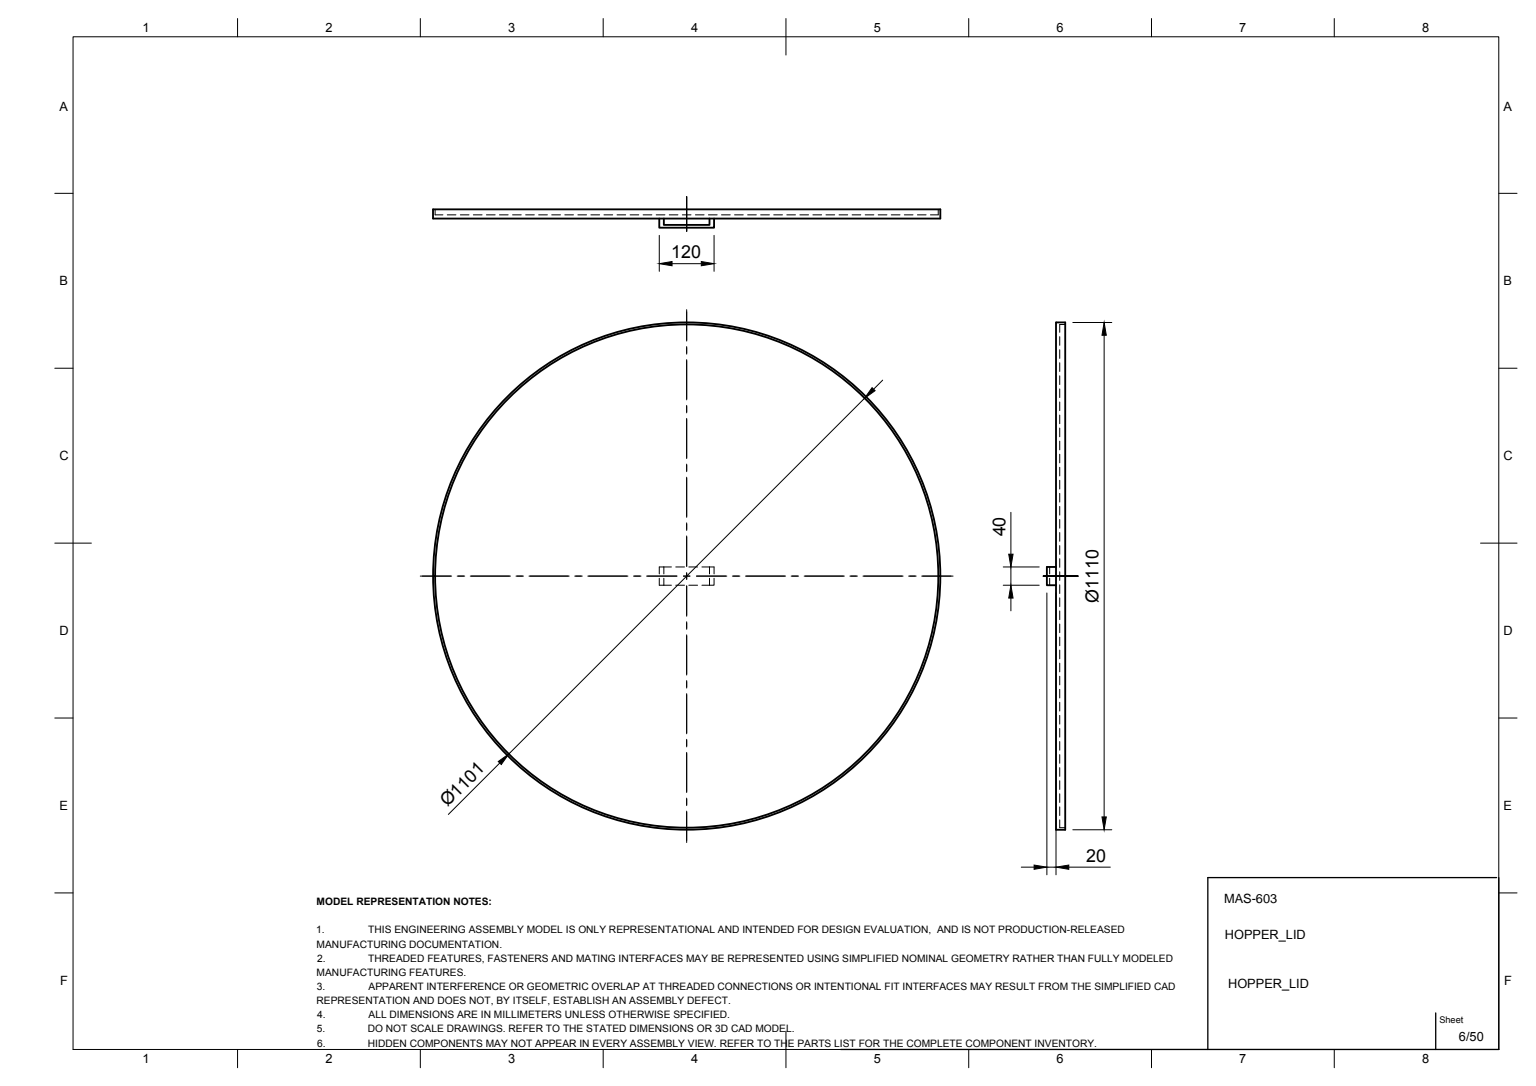
ISO-10303-21;
HEADER;
FILE_DESCRIPTION((''),'2;1');
FILE_NAME('HOPPER_LID.step','2026-10-01T22:06:14-07:00',(''),(''),'','','');
FILE_SCHEMA (('AUTOMOTIVE_DESIGN { 1 0 10303 214 3 1 1 }'));
ENDSEC;
DATA;
#10=MECHANICAL_DESIGN_GEOMETRIC_PRESENTATION_REPRESENTATION('',(#982),#50440);
#892=SHAPE_REPRESENTATION_RELATIONSHIP('SRR','None',#50622,#937) ;
#937=ADVANCED_BREP_SHAPE_REPRESENTATION('',(#1038),#50391) ;
#982=STYLED_ITEM('',(#50884),#1038) ;
#1038=MANIFOLD_SOLID_BREP('HOPPER_LID',#28630) ;
#1127=FACE_BOUND('',#3985,.T.) ;
#1128=FACE_BOUND('',#3989,.T.) ;
#1129=FACE_BOUND('',#3990,.T.) ;
#1467=PLANE('',#29313) ;
#1468=PLANE('',#29314) ;
#1469=PLANE('',#29315) ;
#1470=PLANE('',#29316) ;
#1471=PLANE('',#29317) ;
#1472=PLANE('',#29318) ;
#1473=PLANE('',#29319) ;
#1474=PLANE('',#29320) ;
#1475=PLANE('',#29324) ;
#1476=PLANE('',#29328) ;
#1477=PLANE('',#29329) ;
#2406=FACE_OUTER_BOUND('',#3975,.T.) ;
#2407=FACE_OUTER_BOUND('',#3976,.T.) ;
#2408=FACE_OUTER_BOUND('',#3977,.T.) ;
#2409=FACE_OUTER_BOUND('',#3978,.T.) ;
#2410=FACE_OUTER_BOUND('',#3979,.T.) ;
#2411=FACE_OUTER_BOUND('',#3980,.T.) ;
#2412=FACE_OUTER_BOUND('',#3981,.T.) ;
#2413=FACE_OUTER_BOUND('',#3982,.T.) ;
#2414=FACE_OUTER_BOUND('',#3983,.T.) ;
#2415=FACE_OUTER_BOUND('',#3984,.T.) ;
#2416=FACE_OUTER_BOUND('',#3986,.T.) ;
#2417=FACE_OUTER_BOUND('',#3987,.T.) ;
#2418=FACE_OUTER_BOUND('',#3988,.T.) ;
#3975=EDGE_LOOP('',(#18917,#18918,#18919,#18920)) ;
#3976=EDGE_LOOP('',(#18921,#18922,#18923,#18924)) ;
#3977=EDGE_LOOP('',(#18925,#18926,#18927,#18928)) ;
#3978=EDGE_LOOP('',(#18929,#18930,#18931,#18932,#18933,#18934,#18935,#18936)) ;
#3979=EDGE_LOOP('',(#18937,#18938,#18939,#18940,#18941,#18942,#18943,#18944)) ;
#3980=EDGE_LOOP('',(#18945,#18946,#18947,#18948)) ;
#3981=EDGE_LOOP('',(#18949,#18950,#18951,#18952)) ;
#3982=EDGE_LOOP('',(#18953,#18954,#18955,#18956)) ;
#3983=EDGE_LOOP('',(#18957,#18958,#18959,#18960)) ;
#3984=EDGE_LOOP('',(#18961)) ;
#3985=EDGE_LOOP('',(#18962)) ;
#3986=EDGE_LOOP('',(#18963,#18964,#18965,#18966)) ;
#3987=EDGE_LOOP('',(#18967)) ;
#3988=EDGE_LOOP('',(#18968)) ;
#3989=EDGE_LOOP('',(#18969,#18970,#18971,#18972)) ;
#3990=EDGE_LOOP('',(#18973,#18974,#18975,#18976)) ;
#5859=LINE('',#41599,#8331) ;
#5860=LINE('',#41601,#8332) ;
#5861=LINE('',#41603,#8333) ;
#5862=LINE('',#41604,#8334) ;
#5863=LINE('',#41607,#8335) ;
#5864=LINE('',#41609,#8336) ;
#5865=LINE('',#41610,#8337) ;
#5866=LINE('',#41613,#8338) ;
#5867=LINE('',#41615,#8339) ;
#5868=LINE('',#41616,#8340) ;
#5869=LINE('',#41619,#8341) ;
#5870=LINE('',#41621,#8342) ;
#5871=LINE('',#41623,#8343) ;
#5872=LINE('',#41625,#8344) ;
#5873=LINE('',#41626,#8345) ;
#5874=LINE('',#41629,#8346) ;
#5875=LINE('',#41631,#8347) ;
#5876=LINE('',#41633,#8348) ;
#5877=LINE('',#41635,#8349) ;
#5878=LINE('',#41636,#8350) ;
#5879=LINE('',#41638,#8351) ;
#5880=LINE('',#41639,#8352) ;
#5881=LINE('',#41641,#8353) ;
#5882=LINE('',#41643,#8354) ;
#5883=LINE('',#41648,#8355) ;
#5884=LINE('',#41656,#8356) ;
#8331=VECTOR('',#32712,1.) ;
#8332=VECTOR('',#32713,1.) ;
#8333=VECTOR('',#32714,1.) ;
#8334=VECTOR('',#32715,1.) ;
#8335=VECTOR('',#32718,1.) ;
#8336=VECTOR('',#32719,1.) ;
#8337=VECTOR('',#32720,1.) ;
#8338=VECTOR('',#32723,1.) ;
#8339=VECTOR('',#32724,1.) ;
#8340=VECTOR('',#32725,1.) ;
#8341=VECTOR('',#32728,1.) ;
#8342=VECTOR('',#32729,1.) ;
#8343=VECTOR('',#32730,1.) ;
#8344=VECTOR('',#32731,1.) ;
#8345=VECTOR('',#32732,1.) ;
#8346=VECTOR('',#32735,1.) ;
#8347=VECTOR('',#32736,1.) ;
#8348=VECTOR('',#32737,1.) ;
#8349=VECTOR('',#32738,1.) ;
#8350=VECTOR('',#32739,1.) ;
#8351=VECTOR('',#32742,1.) ;
#8352=VECTOR('',#32743,1.) ;
#8353=VECTOR('',#32746,1.) ;
#8354=VECTOR('',#32749,1.) ;
#8355=VECTOR('',#32754,55.05) ;
#8356=VECTOR('',#32765,55.5) ;
#10720=CIRCLE('',#29322,55.05) ;
#10721=CIRCLE('',#29323,55.05) ;
#10722=CIRCLE('',#29325,55.5) ;
#10723=CIRCLE('',#29327,55.5) ;
#11963=VERTEX_POINT('',#41597) ;
#11964=VERTEX_POINT('',#41598) ;
#11965=VERTEX_POINT('',#41600) ;
#11966=VERTEX_POINT('',#41602) ;
#11967=VERTEX_POINT('',#41606) ;
#11968=VERTEX_POINT('',#41608) ;
#11969=VERTEX_POINT('',#41612) ;
#11970=VERTEX_POINT('',#41614) ;
#11971=VERTEX_POINT('',#41618) ;
#11972=VERTEX_POINT('',#41620) ;
#11973=VERTEX_POINT('',#41622) ;
#11974=VERTEX_POINT('',#41624) ;
#11975=VERTEX_POINT('',#41628) ;
#11976=VERTEX_POINT('',#41630) ;
#11977=VERTEX_POINT('',#41632) ;
#11978=VERTEX_POINT('',#41634) ;
#11979=VERTEX_POINT('',#41645) ;
#11980=VERTEX_POINT('',#41647) ;
#11981=VERTEX_POINT('',#41651) ;
#11982=VERTEX_POINT('',#41654) ;
#14724=EDGE_CURVE('',#11963,#11964,#5859,.T.) ;
#14725=EDGE_CURVE('',#11965,#11963,#5860,.T.) ;
#14726=EDGE_CURVE('',#11966,#11965,#5861,.T.) ;
#14727=EDGE_CURVE('',#11964,#11966,#5862,.T.) ;
#14728=EDGE_CURVE('',#11964,#11967,#5863,.T.) ;
#14729=EDGE_CURVE('',#11968,#11966,#5864,.T.) ;
#14730=EDGE_CURVE('',#11968,#11967,#5865,.T.) ;
#14731=EDGE_CURVE('',#11969,#11963,#5866,.T.) ;
#14732=EDGE_CURVE('',#11969,#11970,#5867,.T.) ;
#14733=EDGE_CURVE('',#11965,#11970,#5868,.T.) ;
#14734=EDGE_CURVE('',#11971,#11967,#5869,.T.) ;
#14735=EDGE_CURVE('',#11972,#11971,#5870,.T.) ;
#14736=EDGE_CURVE('',#11973,#11972,#5871,.T.) ;
#14737=EDGE_CURVE('',#11973,#11974,#5872,.T.) ;
#14738=EDGE_CURVE('',#11969,#11974,#5873,.T.) ;
#14739=EDGE_CURVE('',#11975,#11970,#5874,.T.) ;
#14740=EDGE_CURVE('',#11976,#11975,#5875,.T.) ;
#14741=EDGE_CURVE('',#11977,#11976,#5876,.T.) ;
#14742=EDGE_CURVE('',#11977,#11978,#5877,.T.) ;
#14743=EDGE_CURVE('',#11968,#11978,#5878,.T.) ;
#14744=EDGE_CURVE('',#11976,#11973,#5879,.T.) ;
#14745=EDGE_CURVE('',#11972,#11977,#5880,.T.) ;
#14746=EDGE_CURVE('',#11978,#11971,#5881,.T.) ;
#14747=EDGE_CURVE('',#11974,#11975,#5882,.T.) ;
#14748=EDGE_CURVE('',#11979,#11979,#10720,.T.) ;
#14749=EDGE_CURVE('',#11979,#11980,#5883,.T.) ;
#14750=EDGE_CURVE('',#11980,#11980,#10721,.T.) ;
#14751=EDGE_CURVE('',#11981,#11981,#10722,.T.) ;
#14752=EDGE_CURVE('',#11982,#11982,#10723,.T.) ;
#14753=EDGE_CURVE('',#11982,#11981,#5884,.T.) ;
#18917=ORIENTED_EDGE('',*,*,#14724,.F.) ;
#18918=ORIENTED_EDGE('',*,*,#14725,.F.) ;
#18919=ORIENTED_EDGE('',*,*,#14726,.F.) ;
#18920=ORIENTED_EDGE('',*,*,#14727,.F.) ;
#18921=ORIENTED_EDGE('',*,*,#14728,.F.) ;
#18922=ORIENTED_EDGE('',*,*,#14727,.T.) ;
#18923=ORIENTED_EDGE('',*,*,#14729,.F.) ;
#18924=ORIENTED_EDGE('',*,*,#14730,.T.) ;
#18925=ORIENTED_EDGE('',*,*,#14731,.F.) ;
#18926=ORIENTED_EDGE('',*,*,#14732,.T.) ;
#18927=ORIENTED_EDGE('',*,*,#14733,.F.) ;
#18928=ORIENTED_EDGE('',*,*,#14725,.T.) ;
#18929=ORIENTED_EDGE('',*,*,#14731,.T.) ;
#18930=ORIENTED_EDGE('',*,*,#14724,.T.) ;
#18931=ORIENTED_EDGE('',*,*,#14728,.T.) ;
#18932=ORIENTED_EDGE('',*,*,#14734,.F.) ;
#18933=ORIENTED_EDGE('',*,*,#14735,.F.) ;
#18934=ORIENTED_EDGE('',*,*,#14736,.F.) ;
#18935=ORIENTED_EDGE('',*,*,#14737,.T.) ;
#18936=ORIENTED_EDGE('',*,*,#14738,.F.) ;
#18937=ORIENTED_EDGE('',*,*,#14729,.T.) ;
#18938=ORIENTED_EDGE('',*,*,#14726,.T.) ;
#18939=ORIENTED_EDGE('',*,*,#14733,.T.) ;
#18940=ORIENTED_EDGE('',*,*,#14739,.F.) ;
#18941=ORIENTED_EDGE('',*,*,#14740,.F.) ;
#18942=ORIENTED_EDGE('',*,*,#14741,.F.) ;
#18943=ORIENTED_EDGE('',*,*,#14742,.T.) ;
#18944=ORIENTED_EDGE('',*,*,#14743,.F.) ;
#18945=ORIENTED_EDGE('',*,*,#14744,.T.) ;
#18946=ORIENTED_EDGE('',*,*,#14736,.T.) ;
#18947=ORIENTED_EDGE('',*,*,#14745,.T.) ;
#18948=ORIENTED_EDGE('',*,*,#14741,.T.) ;
#18949=ORIENTED_EDGE('',*,*,#14735,.T.) ;
#18950=ORIENTED_EDGE('',*,*,#14746,.F.) ;
#18951=ORIENTED_EDGE('',*,*,#14742,.F.) ;
#18952=ORIENTED_EDGE('',*,*,#14745,.F.) ;
#18953=ORIENTED_EDGE('',*,*,#14740,.T.) ;
#18954=ORIENTED_EDGE('',*,*,#14747,.F.) ;
#18955=ORIENTED_EDGE('',*,*,#14737,.F.) ;
#18956=ORIENTED_EDGE('',*,*,#14744,.F.) ;
#18957=ORIENTED_EDGE('',*,*,#14748,.F.) ;
#18958=ORIENTED_EDGE('',*,*,#14749,.T.) ;
#18959=ORIENTED_EDGE('',*,*,#14750,.F.) ;
#18960=ORIENTED_EDGE('',*,*,#14749,.F.) ;
#18961=ORIENTED_EDGE('',*,*,#14751,.T.) ;
#18962=ORIENTED_EDGE('',*,*,#14748,.T.) ;
#18963=ORIENTED_EDGE('',*,*,#14752,.F.) ;
#18964=ORIENTED_EDGE('',*,*,#14753,.T.) ;
#18965=ORIENTED_EDGE('',*,*,#14751,.F.) ;
#18966=ORIENTED_EDGE('',*,*,#14753,.F.) ;
#18967=ORIENTED_EDGE('',*,*,#14750,.T.) ;
#18968=ORIENTED_EDGE('',*,*,#14752,.T.) ;
#18969=ORIENTED_EDGE('',*,*,#14738,.T.) ;
#18970=ORIENTED_EDGE('',*,*,#14747,.T.) ;
#18971=ORIENTED_EDGE('',*,*,#14739,.T.) ;
#18972=ORIENTED_EDGE('',*,*,#14732,.F.) ;
#18973=ORIENTED_EDGE('',*,*,#14730,.F.) ;
#18974=ORIENTED_EDGE('',*,*,#14743,.T.) ;
#18975=ORIENTED_EDGE('',*,*,#14746,.T.) ;
#18976=ORIENTED_EDGE('',*,*,#14734,.T.) ;
#26656=CYLINDRICAL_SURFACE('',#29321,55.05) ;
#26657=CYLINDRICAL_SURFACE('',#29326,55.5) ;
#27141=ADVANCED_FACE('',(#2406),#1467,.F.) ;
#27142=ADVANCED_FACE('',(#2407),#1468,.T.) ;
#27143=ADVANCED_FACE('',(#2408),#1469,.T.) ;
#27144=ADVANCED_FACE('',(#2409),#1470,.F.) ;
#27145=ADVANCED_FACE('',(#2410),#1471,.F.) ;
#27146=ADVANCED_FACE('',(#2411),#1472,.T.) ;
#27147=ADVANCED_FACE('',(#2412),#1473,.F.) ;
#27148=ADVANCED_FACE('',(#2413),#1474,.F.) ;
#27149=ADVANCED_FACE('',(#2414),#26656,.F.) ;
#27150=ADVANCED_FACE('',(#2415,#1127),#1475,.T.) ;
#27151=ADVANCED_FACE('',(#2416),#26657,.T.) ;
#27152=ADVANCED_FACE('',(#2417),#1476,.T.) ;
#27153=ADVANCED_FACE('',(#2418,#1128,#1129),#1477,.T.) ;
#28630=CLOSED_SHELL('',(#27141,#27142,#27143,#27144,#27145,#27146,#27147,
#27148,#27149,#27150,#27151,#27152,#27153)) ;
#29312=AXIS2_PLACEMENT_3D('',#41595,#32708,#32709) ;
#29313=AXIS2_PLACEMENT_3D('',#41596,#32710,#32711) ;
#29314=AXIS2_PLACEMENT_3D('',#41605,#32716,#32717) ;
#29315=AXIS2_PLACEMENT_3D('',#41611,#32721,#32722) ;
#29316=AXIS2_PLACEMENT_3D('',#41617,#32726,#32727) ;
#29317=AXIS2_PLACEMENT_3D('',#41627,#32733,#32734) ;
#29318=AXIS2_PLACEMENT_3D('',#41637,#32740,#32741) ;
#29319=AXIS2_PLACEMENT_3D('',#41640,#32744,#32745) ;
#29320=AXIS2_PLACEMENT_3D('',#41642,#32747,#32748) ;
#29321=AXIS2_PLACEMENT_3D('',#41644,#32750,#32751) ;
#29322=AXIS2_PLACEMENT_3D('',#41646,#32752,#32753) ;
#29323=AXIS2_PLACEMENT_3D('',#41649,#32755,#32756) ;
#29324=AXIS2_PLACEMENT_3D('',#41650,#32757,#32758) ;
#29325=AXIS2_PLACEMENT_3D('',#41652,#32759,#32760) ;
#29326=AXIS2_PLACEMENT_3D('',#41653,#32761,#32762) ;
#29327=AXIS2_PLACEMENT_3D('',#41655,#32763,#32764) ;
#29328=AXIS2_PLACEMENT_3D('',#41657,#32766,#32767) ;
#29329=AXIS2_PLACEMENT_3D('',#41658,#32768,#32769) ;
#32708=DIRECTION('axis',(0.,0.,1.)) ;
#32709=DIRECTION('refdir',(1.,0.,0.)) ;
#32710=DIRECTION('center_axis',(0.,0.,1.)) ;
#32711=DIRECTION('ref_axis',(1.,0.,0.)) ;
#32712=DIRECTION('',(-1.,0.,0.)) ;
#32713=DIRECTION('',(0.,1.,0.)) ;
#32714=DIRECTION('',(1.,0.,0.)) ;
#32715=DIRECTION('',(0.,-1.,0.)) ;
#32716=DIRECTION('center_axis',(1.,0.,0.)) ;
#32717=DIRECTION('ref_axis',(0.,0.,-1.)) ;
#32718=DIRECTION('',(0.,0.,-1.)) ;
#32719=DIRECTION('',(0.,0.,1.)) ;
#32720=DIRECTION('',(0.,1.,0.)) ;
#32721=DIRECTION('center_axis',(-1.,0.,0.)) ;
#32722=DIRECTION('ref_axis',(0.,0.,1.)) ;
#32723=DIRECTION('',(0.,0.,1.)) ;
#32724=DIRECTION('',(0.,-1.,0.)) ;
#32725=DIRECTION('',(0.,0.,-1.)) ;
#32726=DIRECTION('center_axis',(0.,-1.,0.)) ;
#32727=DIRECTION('ref_axis',(0.,0.,-1.)) ;
#32728=DIRECTION('',(1.,0.,0.)) ;
#32729=DIRECTION('',(0.,0.,-1.)) ;
#32730=DIRECTION('',(-1.,0.,0.)) ;
#32731=DIRECTION('',(0.,0.,-1.)) ;
#32732=DIRECTION('',(1.,0.,0.)) ;
#32733=DIRECTION('center_axis',(0.,1.,0.)) ;
#32734=DIRECTION('ref_axis',(0.,0.,1.)) ;
#32735=DIRECTION('',(-1.,0.,0.)) ;
#32736=DIRECTION('',(0.,0.,-1.)) ;
#32737=DIRECTION('',(1.,0.,0.)) ;
#32738=DIRECTION('',(0.,0.,-1.)) ;
#32739=DIRECTION('',(-1.,0.,0.)) ;
#32740=DIRECTION('center_axis',(0.,0.,1.)) ;
#32741=DIRECTION('ref_axis',(1.,0.,0.)) ;
#32742=DIRECTION('',(0.,1.,0.)) ;
#32743=DIRECTION('',(0.,-1.,0.)) ;
#32744=DIRECTION('center_axis',(1.,0.,0.)) ;
#32745=DIRECTION('ref_axis',(0.,0.,-1.)) ;
#32746=DIRECTION('',(0.,1.,0.)) ;
#32747=DIRECTION('center_axis',(-1.,0.,0.)) ;
#32748=DIRECTION('ref_axis',(0.,0.,1.)) ;
#32749=DIRECTION('',(0.,-1.,0.)) ;
#32750=DIRECTION('center_axis',(0.,0.,1.)) ;
#32751=DIRECTION('ref_axis',(1.,0.,0.)) ;
#32752=DIRECTION('center_axis',(0.,0.,1.)) ;
#32753=DIRECTION('ref_axis',(1.,0.,0.)) ;
#32754=DIRECTION('',(0.,0.,1.)) ;
#32755=DIRECTION('center_axis',(0.,0.,-1.)) ;
#32756=DIRECTION('ref_axis',(1.,0.,0.)) ;
#32757=DIRECTION('center_axis',(0.,0.,-1.)) ;
#32758=DIRECTION('ref_axis',(-1.,0.,0.)) ;
#32759=DIRECTION('center_axis',(0.,0.,-1.)) ;
#32760=DIRECTION('ref_axis',(1.,0.,0.)) ;
#32761=DIRECTION('center_axis',(0.,0.,1.)) ;
#32762=DIRECTION('ref_axis',(1.,0.,0.)) ;
#32763=DIRECTION('center_axis',(0.,0.,1.)) ;
#32764=DIRECTION('ref_axis',(1.,0.,0.)) ;
#32765=DIRECTION('',(0.,0.,-1.)) ;
#32766=DIRECTION('center_axis',(0.,0.,-1.)) ;
#32767=DIRECTION('ref_axis',(-1.,0.,0.)) ;
#32768=DIRECTION('center_axis',(0.,0.,1.)) ;
#32769=DIRECTION('ref_axis',(1.,0.,0.)) ;
#41595=CARTESIAN_POINT('',(0.,0.,0.)) ;
#41596=CARTESIAN_POINT('Origin',(0.,0.,113.4)) ;
#41597=CARTESIAN_POINT('',(5.,2.,113.4)) ;
#41598=CARTESIAN_POINT('',(-5.,2.,113.4)) ;
#41599=CARTESIAN_POINT('',(0.,2.,113.4)) ;
#41600=CARTESIAN_POINT('',(5.,-2.,113.4)) ;
#41601=CARTESIAN_POINT('',(5.,0.,113.4)) ;
#41602=CARTESIAN_POINT('',(-5.,-2.,113.4)) ;
#41603=CARTESIAN_POINT('',(0.,-2.,113.4)) ;
#41604=CARTESIAN_POINT('',(-5.,0.,113.4)) ;
#41605=CARTESIAN_POINT('Origin',(-5.,0.,112.7)) ;
#41606=CARTESIAN_POINT('',(-5.,2.,112.)) ;
#41607=CARTESIAN_POINT('',(-5.,2.,112.85)) ;
#41608=CARTESIAN_POINT('',(-5.,-2.,112.)) ;
#41609=CARTESIAN_POINT('',(-5.,-2.,112.85)) ;
#41610=CARTESIAN_POINT('',(-5.,0.,112.)) ;
#41611=CARTESIAN_POINT('Origin',(5.,0.,112.7)) ;
#41612=CARTESIAN_POINT('',(5.,2.,112.)) ;
#41613=CARTESIAN_POINT('',(5.,2.,112.85)) ;
#41614=CARTESIAN_POINT('',(5.,-2.,112.)) ;
#41615=CARTESIAN_POINT('',(5.,0.,112.)) ;
#41616=CARTESIAN_POINT('',(5.,-2.,112.85)) ;
#41617=CARTESIAN_POINT('Origin',(0.,2.,113.)) ;
#41618=CARTESIAN_POINT('',(-6.,2.,112.)) ;
#41619=CARTESIAN_POINT('',(0.,2.,112.)) ;
#41620=CARTESIAN_POINT('',(-6.,2.,114.)) ;
#41621=CARTESIAN_POINT('',(-6.,2.,113.)) ;
#41622=CARTESIAN_POINT('',(6.,2.,114.)) ;
#41623=CARTESIAN_POINT('',(0.,2.,114.)) ;
#41624=CARTESIAN_POINT('',(6.,2.,112.)) ;
#41625=CARTESIAN_POINT('',(6.,2.,113.)) ;
#41626=CARTESIAN_POINT('',(0.,2.,112.)) ;
#41627=CARTESIAN_POINT('Origin',(0.,-2.,113.)) ;
#41628=CARTESIAN_POINT('',(6.,-2.,112.)) ;
#41629=CARTESIAN_POINT('',(0.,-2.,112.)) ;
#41630=CARTESIAN_POINT('',(6.,-2.,114.)) ;
#41631=CARTESIAN_POINT('',(6.,-2.,113.)) ;
#41632=CARTESIAN_POINT('',(-6.,-2.,114.)) ;
#41633=CARTESIAN_POINT('',(0.,-2.,114.)) ;
#41634=CARTESIAN_POINT('',(-6.,-2.,112.)) ;
#41635=CARTESIAN_POINT('',(-6.,-2.,113.)) ;
#41636=CARTESIAN_POINT('',(0.,-2.,112.)) ;
#41637=CARTESIAN_POINT('Origin',(0.,0.,114.)) ;
#41638=CARTESIAN_POINT('',(6.,0.,114.)) ;
#41639=CARTESIAN_POINT('',(-6.,0.,114.)) ;
#41640=CARTESIAN_POINT('Origin',(-6.,0.,113.)) ;
#41641=CARTESIAN_POINT('',(-6.,0.,112.)) ;
#41642=CARTESIAN_POINT('Origin',(6.,0.,113.)) ;
#41643=CARTESIAN_POINT('',(6.,0.,112.)) ;
#41644=CARTESIAN_POINT('Origin',(0.,0.,110.6)) ;
#41645=CARTESIAN_POINT('',(-55.05,-6.74168062930618E-15,110.)) ;
#41646=CARTESIAN_POINT('Origin',(0.,0.,110.)) ;
#41647=CARTESIAN_POINT('',(-55.05,6.74168062930618E-15,111.2)) ;
#41648=CARTESIAN_POINT('',(-55.05,-6.74168062930618E-15,110.6)) ;
#41649=CARTESIAN_POINT('Origin',(0.,0.,111.2)) ;
#41650=CARTESIAN_POINT('Origin',(0.,0.,110.)) ;
#41651=CARTESIAN_POINT('',(-55.5,-6.79678973526781E-15,110.)) ;
#41652=CARTESIAN_POINT('Origin',(0.,0.,110.)) ;
#41653=CARTESIAN_POINT('Origin',(0.,0.,111.6)) ;
#41654=CARTESIAN_POINT('',(-55.5,-6.79678973526781E-15,112.)) ;
#41655=CARTESIAN_POINT('Origin',(0.,0.,112.)) ;
#41656=CARTESIAN_POINT('',(-55.5,-6.79678973526781E-15,111.6)) ;
#41657=CARTESIAN_POINT('Origin',(0.,0.,111.2)) ;
#41658=CARTESIAN_POINT('Origin',(0.,0.,112.)) ;
#50338=UNCERTAINTY_MEASURE_WITH_UNIT(LENGTH_MEASURE(0.001),#50441,
'DISTANCE_ACCURACY_VALUE',
'Maximum model space distance between geometric entities at asserted c
onnectivities') ;
#50387=UNCERTAINTY_MEASURE_WITH_UNIT(LENGTH_MEASURE(0.001),#50441,
'DISTANCE_ACCURACY_VALUE',
'Maximum model space distance between geometric entities at asserted c
onnectivities') ;
#50391=(
GEOMETRIC_REPRESENTATION_CONTEXT(3)
GLOBAL_UNCERTAINTY_ASSIGNED_CONTEXT((#50338))
GLOBAL_UNIT_ASSIGNED_CONTEXT((#50441,#50443,#50444))
REPRESENTATION_CONTEXT('','3D')
) ;
#50440=(
GEOMETRIC_REPRESENTATION_CONTEXT(3)
GLOBAL_UNCERTAINTY_ASSIGNED_CONTEXT((#50387))
GLOBAL_UNIT_ASSIGNED_CONTEXT((#50441,#50443,#50444))
REPRESENTATION_CONTEXT('','3D')
) ;
#50441=(
LENGTH_UNIT()
NAMED_UNIT(*)
SI_UNIT(.CENTI.,.METRE.)
) ;
#50443=(
NAMED_UNIT(*)
PLANE_ANGLE_UNIT()
SI_UNIT($,.RADIAN.)
) ;
#50444=(
NAMED_UNIT(*)
SI_UNIT($,.STERADIAN.)
SOLID_ANGLE_UNIT()
) ;
#50448=SHAPE_DEFINITION_REPRESENTATION(#50500,#50622) ;
#50500=PRODUCT_DEFINITION_SHAPE('',$,#50675) ;
#50622=SHAPE_REPRESENTATION('',(#29312),#50391) ;
#50671=PRODUCT_DEFINITION_CONTEXT('part definition',#50829,'design') ;
#50675=PRODUCT_DEFINITION('HOPPER_LID','HOPPER_LID',#50727,
#50671) ;
#50727=PRODUCT_DEFINITION_FORMATION('',$,#50834) ;
#50829=APPLICATION_CONTEXT(
'Core Data for Automotive Mechanical Design Process') ;
#50830=PRODUCT_CONTEXT('part definition',#50829,'mechanical') ;
#50834=PRODUCT('HOPPER_LID','HOPPER_LID',$,(#50830)) ;
#50884=PRESENTATION_STYLE_ASSIGNMENT((#50891)) ;
#50891=SURFACE_STYLE_USAGE(.BOTH.,#50898) ;
#50898=SURFACE_SIDE_STYLE('',(#50905)) ;
#50905=SURFACE_STYLE_FILL_AREA(#50912) ;
#50912=FILL_AREA_STYLE('Surface - Matte',(#50919)) ;
#50919=FILL_AREA_STYLE_COLOUR('Surface - Matte',#50926) ;
#50926=COLOUR_RGB('Surface - Matte', 0.72549020, 0.75294118, 0.79215686) ;
ENDSEC;
END-ISO-10303-21;
